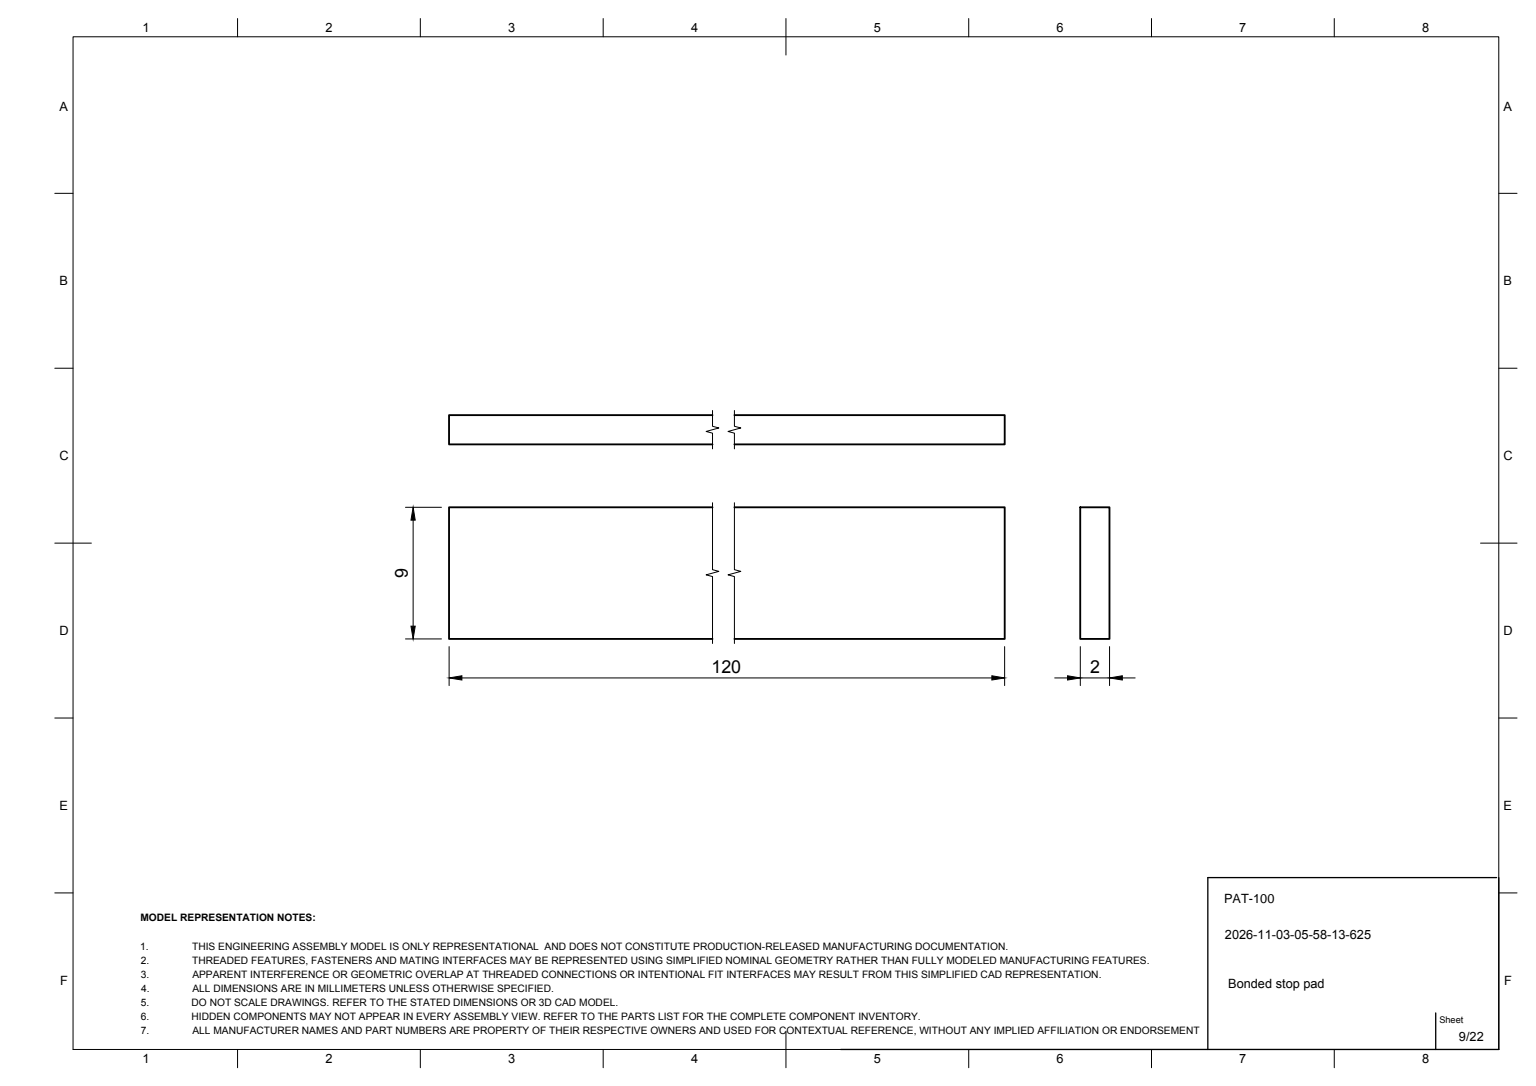
ISO-10303-21;
HEADER;
/* Generated by software containing ST-Developer
 * from STEP Tools, Inc. (www.steptools.com) 
 */

FILE_DESCRIPTION(
/* description */ (''),
/* implementation_level */ '2;1');

FILE_NAME(
/* name */ 'Bonded stop pad.step',
/* time_stamp */ '2026-10-29T16:43:51-07:00',
/* author */ (''),
/* organization */ (''),
/* preprocessor_version */ 'ST-DEVELOPER v20.2',
/* originating_system */ 'Autodesk Translation Framework v15.17.0.0',
/* authorisation */ '');

FILE_SCHEMA (('AUTOMOTIVE_DESIGN { 1 0 10303 214 3 1 1 }'));
ENDSEC;

DATA;
#10=MECHANICAL_DESIGN_GEOMETRIC_PRESENTATION_REPRESENTATION('',(#370),#10292);
#324=SHAPE_REPRESENTATION_RELATIONSHIP('SRR','None',#10420,#347);
#347=ADVANCED_BREP_SHAPE_REPRESENTATION('',(#392),#10272);
#370=STYLED_ITEM('',(#10642),#392);
#392=MANIFOLD_SOLID_BREP('Body1',#5013);
#574=PLANE('',#5440);
#575=PLANE('',#5441);
#576=PLANE('',#5442);
#577=PLANE('',#5443);
#578=PLANE('',#5444);
#579=PLANE('',#5445);
#788=FACE_OUTER_BOUND('',#1125,.T.);
#789=FACE_OUTER_BOUND('',#1126,.T.);
#790=FACE_OUTER_BOUND('',#1127,.T.);
#791=FACE_OUTER_BOUND('',#1128,.T.);
#792=FACE_OUTER_BOUND('',#1129,.T.);
#793=FACE_OUTER_BOUND('',#1130,.T.);
#1125=EDGE_LOOP('',(#3777,#3778,#3779,#3780));
#1126=EDGE_LOOP('',(#3781,#3782,#3783,#3784));
#1127=EDGE_LOOP('',(#3785,#3786,#3787,#3788));
#1128=EDGE_LOOP('',(#3789,#3790,#3791,#3792));
#1129=EDGE_LOOP('',(#3793,#3794,#3795,#3796));
#1130=EDGE_LOOP('',(#3797,#3798,#3799,#3800));
#1530=LINE('',#7800,#1922);
#1531=LINE('',#7802,#1923);
#1532=LINE('',#7804,#1924);
#1533=LINE('',#7805,#1925);
#1534=LINE('',#7808,#1926);
#1535=LINE('',#7810,#1927);
#1536=LINE('',#7811,#1928);
#1537=LINE('',#7814,#1929);
#1538=LINE('',#7816,#1930);
#1539=LINE('',#7817,#1931);
#1540=LINE('',#7819,#1932);
#1541=LINE('',#7820,#1933);
#1922=VECTOR('',#6287,1.);
#1923=VECTOR('',#6288,1.);
#1924=VECTOR('',#6289,1.);
#1925=VECTOR('',#6290,1.);
#1926=VECTOR('',#6293,1.);
#1927=VECTOR('',#6294,1.);
#1928=VECTOR('',#6295,1.);
#1929=VECTOR('',#6298,1.);
#1930=VECTOR('',#6299,1.);
#1931=VECTOR('',#6300,1.);
#1932=VECTOR('',#6303,1.);
#1933=VECTOR('',#6304,1.);
#2515=VERTEX_POINT('',#7798);
#2516=VERTEX_POINT('',#7799);
#2517=VERTEX_POINT('',#7801);
#2518=VERTEX_POINT('',#7803);
#2519=VERTEX_POINT('',#7807);
#2520=VERTEX_POINT('',#7809);
#2521=VERTEX_POINT('',#7813);
#2522=VERTEX_POINT('',#7815);
#2979=EDGE_CURVE('',#2515,#2516,#1530,.T.);
#2980=EDGE_CURVE('',#2516,#2517,#1531,.T.);
#2981=EDGE_CURVE('',#2518,#2517,#1532,.T.);
#2982=EDGE_CURVE('',#2515,#2518,#1533,.T.);
#2983=EDGE_CURVE('',#2519,#2515,#1534,.T.);
#2984=EDGE_CURVE('',#2520,#2518,#1535,.T.);
#2985=EDGE_CURVE('',#2519,#2520,#1536,.T.);
#2986=EDGE_CURVE('',#2521,#2519,#1537,.T.);
#2987=EDGE_CURVE('',#2522,#2520,#1538,.T.);
#2988=EDGE_CURVE('',#2521,#2522,#1539,.T.);
#2989=EDGE_CURVE('',#2516,#2521,#1540,.T.);
#2990=EDGE_CURVE('',#2517,#2522,#1541,.T.);
#3777=ORIENTED_EDGE('',*,*,#2979,.T.);
#3778=ORIENTED_EDGE('',*,*,#2980,.T.);
#3779=ORIENTED_EDGE('',*,*,#2981,.F.);
#3780=ORIENTED_EDGE('',*,*,#2982,.F.);
#3781=ORIENTED_EDGE('',*,*,#2983,.T.);
#3782=ORIENTED_EDGE('',*,*,#2982,.T.);
#3783=ORIENTED_EDGE('',*,*,#2984,.F.);
#3784=ORIENTED_EDGE('',*,*,#2985,.F.);
#3785=ORIENTED_EDGE('',*,*,#2986,.T.);
#3786=ORIENTED_EDGE('',*,*,#2985,.T.);
#3787=ORIENTED_EDGE('',*,*,#2987,.F.);
#3788=ORIENTED_EDGE('',*,*,#2988,.F.);
#3789=ORIENTED_EDGE('',*,*,#2989,.T.);
#3790=ORIENTED_EDGE('',*,*,#2988,.T.);
#3791=ORIENTED_EDGE('',*,*,#2990,.F.);
#3792=ORIENTED_EDGE('',*,*,#2980,.F.);
#3793=ORIENTED_EDGE('',*,*,#2990,.T.);
#3794=ORIENTED_EDGE('',*,*,#2987,.T.);
#3795=ORIENTED_EDGE('',*,*,#2984,.T.);
#3796=ORIENTED_EDGE('',*,*,#2981,.T.);
#3797=ORIENTED_EDGE('',*,*,#2989,.F.);
#3798=ORIENTED_EDGE('',*,*,#2979,.F.);
#3799=ORIENTED_EDGE('',*,*,#2983,.F.);
#3800=ORIENTED_EDGE('',*,*,#2986,.F.);
#4797=ADVANCED_FACE('',(#788),#574,.T.);
#4798=ADVANCED_FACE('',(#789),#575,.T.);
#4799=ADVANCED_FACE('',(#790),#576,.T.);
#4800=ADVANCED_FACE('',(#791),#577,.T.);
#4801=ADVANCED_FACE('',(#792),#578,.T.);
#4802=ADVANCED_FACE('',(#793),#579,.F.);
#5013=CLOSED_SHELL('',(#4797,#4798,#4799,#4800,#4801,#4802));
#5439=AXIS2_PLACEMENT_3D('',#7796,#6283,#6284);
#5440=AXIS2_PLACEMENT_3D('',#7797,#6285,#6286);
#5441=AXIS2_PLACEMENT_3D('',#7806,#6291,#6292);
#5442=AXIS2_PLACEMENT_3D('',#7812,#6296,#6297);
#5443=AXIS2_PLACEMENT_3D('',#7818,#6301,#6302);
#5444=AXIS2_PLACEMENT_3D('',#7821,#6305,#6306);
#5445=AXIS2_PLACEMENT_3D('',#7822,#6307,#6308);
#6283=DIRECTION('axis',(0.,0.,1.));
#6284=DIRECTION('refdir',(1.,0.,0.));
#6285=DIRECTION('center_axis',(0.,1.,0.));
#6286=DIRECTION('ref_axis',(-1.,0.,0.));
#6287=DIRECTION('',(-1.,0.,0.));
#6288=DIRECTION('',(0.,0.,1.));
#6289=DIRECTION('',(-1.,0.,0.));
#6290=DIRECTION('',(0.,0.,1.));
#6291=DIRECTION('center_axis',(1.,0.,0.));
#6292=DIRECTION('ref_axis',(0.,1.,0.));
#6293=DIRECTION('',(0.,1.,0.));
#6294=DIRECTION('',(0.,1.,0.));
#6295=DIRECTION('',(0.,0.,1.));
#6296=DIRECTION('center_axis',(0.,-1.,0.));
#6297=DIRECTION('ref_axis',(1.,0.,0.));
#6298=DIRECTION('',(1.,0.,0.));
#6299=DIRECTION('',(1.,0.,0.));
#6300=DIRECTION('',(0.,0.,1.));
#6301=DIRECTION('center_axis',(-1.,0.,0.));
#6302=DIRECTION('ref_axis',(0.,-1.,0.));
#6303=DIRECTION('',(0.,-1.,0.));
#6304=DIRECTION('',(0.,-1.,0.));
#6305=DIRECTION('center_axis',(0.,0.,1.));
#6306=DIRECTION('ref_axis',(1.,0.,0.));
#6307=DIRECTION('center_axis',(0.,0.,1.));
#6308=DIRECTION('ref_axis',(1.,0.,0.));
#7796=CARTESIAN_POINT('',(0.,0.,0.));
#7797=CARTESIAN_POINT('Origin',(4.2,6.,1.6));
#7798=CARTESIAN_POINT('',(4.2,6.,1.6));
#7799=CARTESIAN_POINT('',(4.,6.,1.6));
#7800=CARTESIAN_POINT('',(4.2,6.,1.6));
#7801=CARTESIAN_POINT('',(4.,6.,2.5));
#7802=CARTESIAN_POINT('',(4.,6.,1.6));
#7803=CARTESIAN_POINT('',(4.2,6.,2.5));
#7804=CARTESIAN_POINT('',(4.2,6.,2.5));
#7805=CARTESIAN_POINT('',(4.2,6.,1.6));
#7806=CARTESIAN_POINT('Origin',(4.2,-6.,1.6));
#7807=CARTESIAN_POINT('',(4.2,-6.,1.6));
#7808=CARTESIAN_POINT('',(4.2,-6.,1.6));
#7809=CARTESIAN_POINT('',(4.2,-6.,2.5));
#7810=CARTESIAN_POINT('',(4.2,-6.,2.5));
#7811=CARTESIAN_POINT('',(4.2,-6.,1.6));
#7812=CARTESIAN_POINT('Origin',(4.,-6.,1.6));
#7813=CARTESIAN_POINT('',(4.,-6.,1.6));
#7814=CARTESIAN_POINT('',(4.,-6.,1.6));
#7815=CARTESIAN_POINT('',(4.,-6.,2.5));
#7816=CARTESIAN_POINT('',(4.,-6.,2.5));
#7817=CARTESIAN_POINT('',(4.,-6.,1.6));
#7818=CARTESIAN_POINT('Origin',(4.,6.,1.6));
#7819=CARTESIAN_POINT('',(4.,6.,1.6));
#7820=CARTESIAN_POINT('',(4.,6.,2.5));
#7821=CARTESIAN_POINT('Origin',(4.1,0.,2.5));
#7822=CARTESIAN_POINT('Origin',(4.1,0.,1.6));
#10244=UNCERTAINTY_MEASURE_WITH_UNIT(LENGTH_MEASURE(0.001),#10293,
'DISTANCE_ACCURACY_VALUE',
'Maximum model space distance between geometric entities at asserted c
onnectivities');
#10264=UNCERTAINTY_MEASURE_WITH_UNIT(LENGTH_MEASURE(0.001),#10293,
'DISTANCE_ACCURACY_VALUE',
'Maximum model space distance between geometric entities at asserted c
onnectivities');
#10272=(
GEOMETRIC_REPRESENTATION_CONTEXT(3)
GLOBAL_UNCERTAINTY_ASSIGNED_CONTEXT((#10244))
GLOBAL_UNIT_ASSIGNED_CONTEXT((#10293,#10295,#10296))
REPRESENTATION_CONTEXT('','3D')
);
#10292=(
GEOMETRIC_REPRESENTATION_CONTEXT(3)
GLOBAL_UNCERTAINTY_ASSIGNED_CONTEXT((#10264))
GLOBAL_UNIT_ASSIGNED_CONTEXT((#10293,#10295,#10296))
REPRESENTATION_CONTEXT('','3D')
);
#10293=(
LENGTH_UNIT()
NAMED_UNIT(*)
SI_UNIT(.CENTI.,.METRE.)
);
#10295=(
NAMED_UNIT(*)
PLANE_ANGLE_UNIT()
SI_UNIT($,.RADIAN.)
);
#10296=(
NAMED_UNIT(*)
SI_UNIT($,.STERADIAN.)
SOLID_ANGLE_UNIT()
);
#10304=SHAPE_DEFINITION_REPRESENTATION(#10331,#10420);
#10331=PRODUCT_DEFINITION_SHAPE('',$,#10448);
#10420=SHAPE_REPRESENTATION('',(#5439),#10272);
#10440=PRODUCT_DEFINITION_CONTEXT('part definition',#10523,'design');
#10448=PRODUCT_DEFINITION('Bonded stop pad','Bonded stop pad',#10475,
#10440);
#10475=PRODUCT_DEFINITION_FORMATION('',$,#10532);
#10523=APPLICATION_CONTEXT(
'Core Data for Automotive Mechanical Design Process');
#10524=PRODUCT_CONTEXT('part definition',#10523,'mechanical');
#10532=PRODUCT('Bonded stop pad','Bonded stop pad',
'Bonded stop pad',(#10524));
#10636=COLOUR_RGB('Off White',0.89,0.88,0.83);
#10637=FILL_AREA_STYLE_COLOUR('',#10636);
#10638=FILL_AREA_STYLE('',(#10637));
#10639=SURFACE_STYLE_FILL_AREA(#10638);
#10640=SURFACE_SIDE_STYLE('',(#10639));
#10641=SURFACE_STYLE_USAGE(.BOTH.,#10640);
#10642=PRESENTATION_STYLE_ASSIGNMENT((#10641));
ENDSEC;
END-ISO-10303-21;
